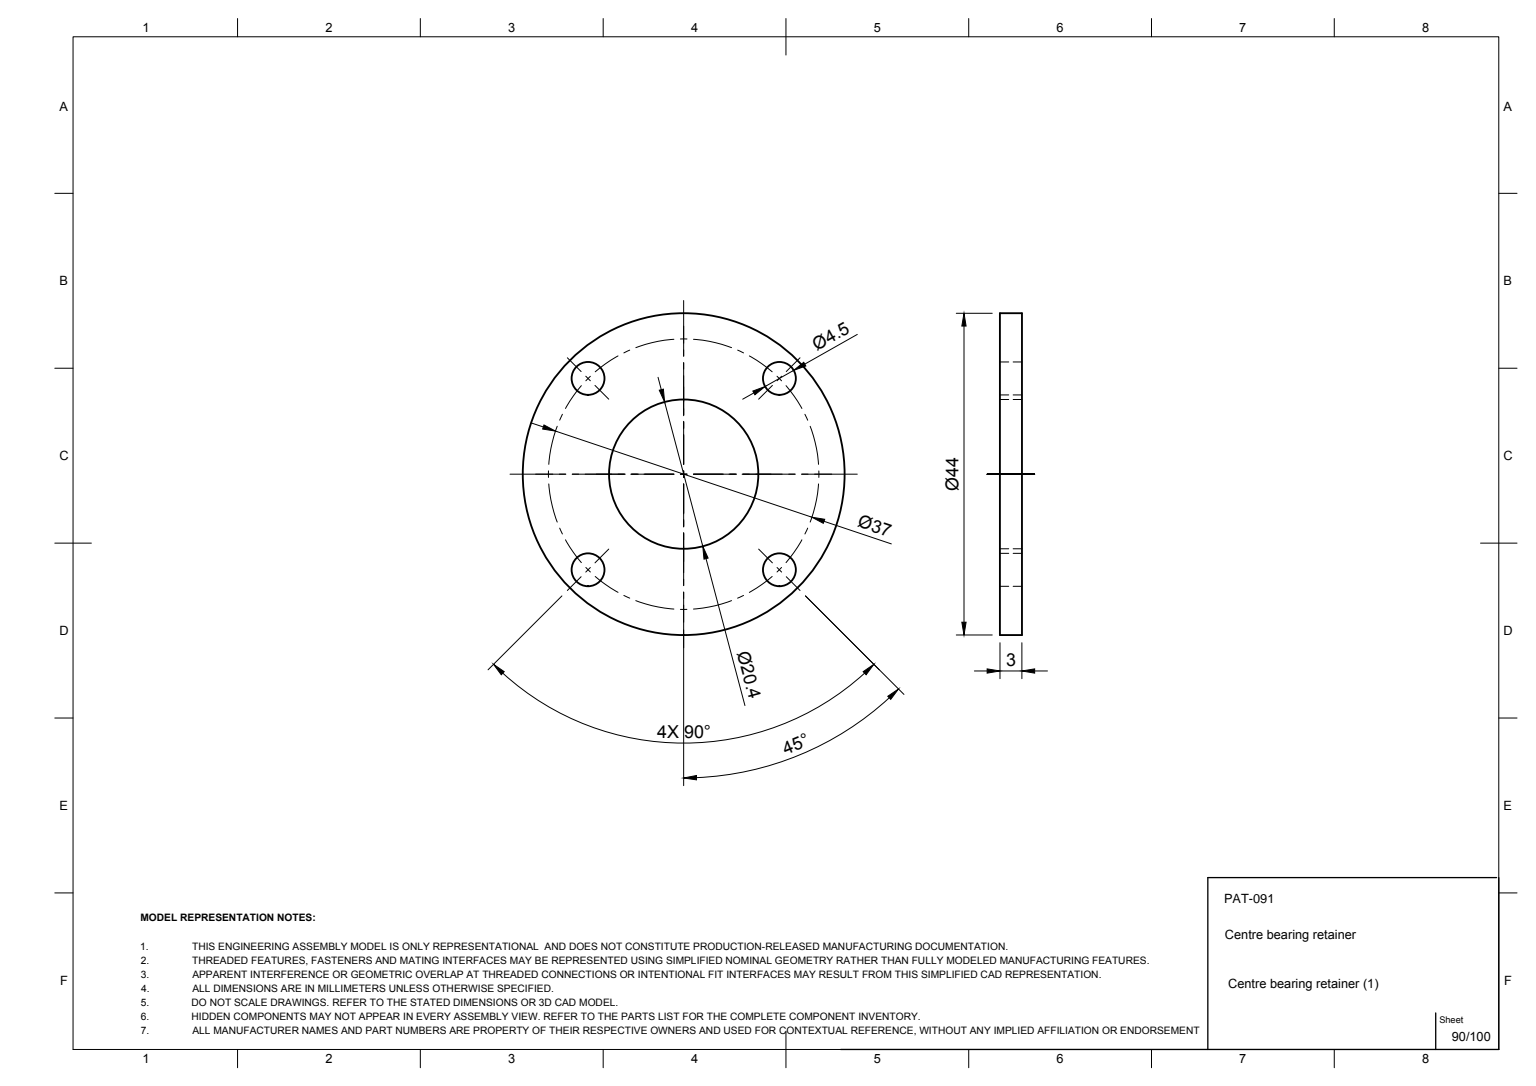
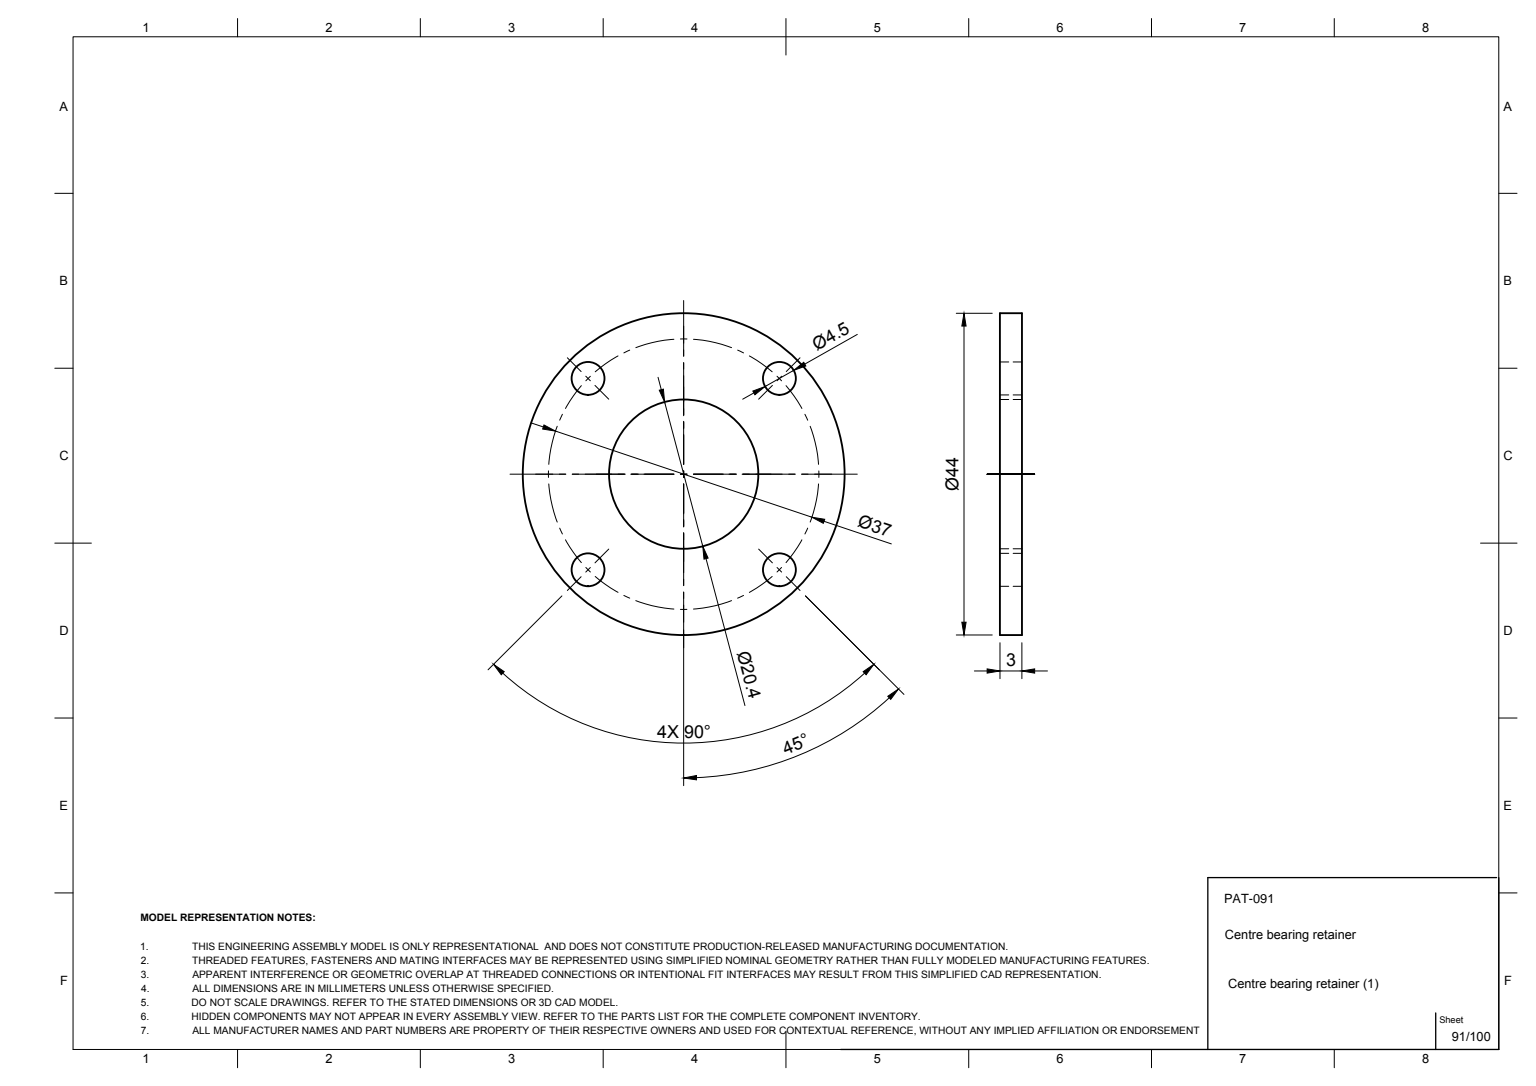
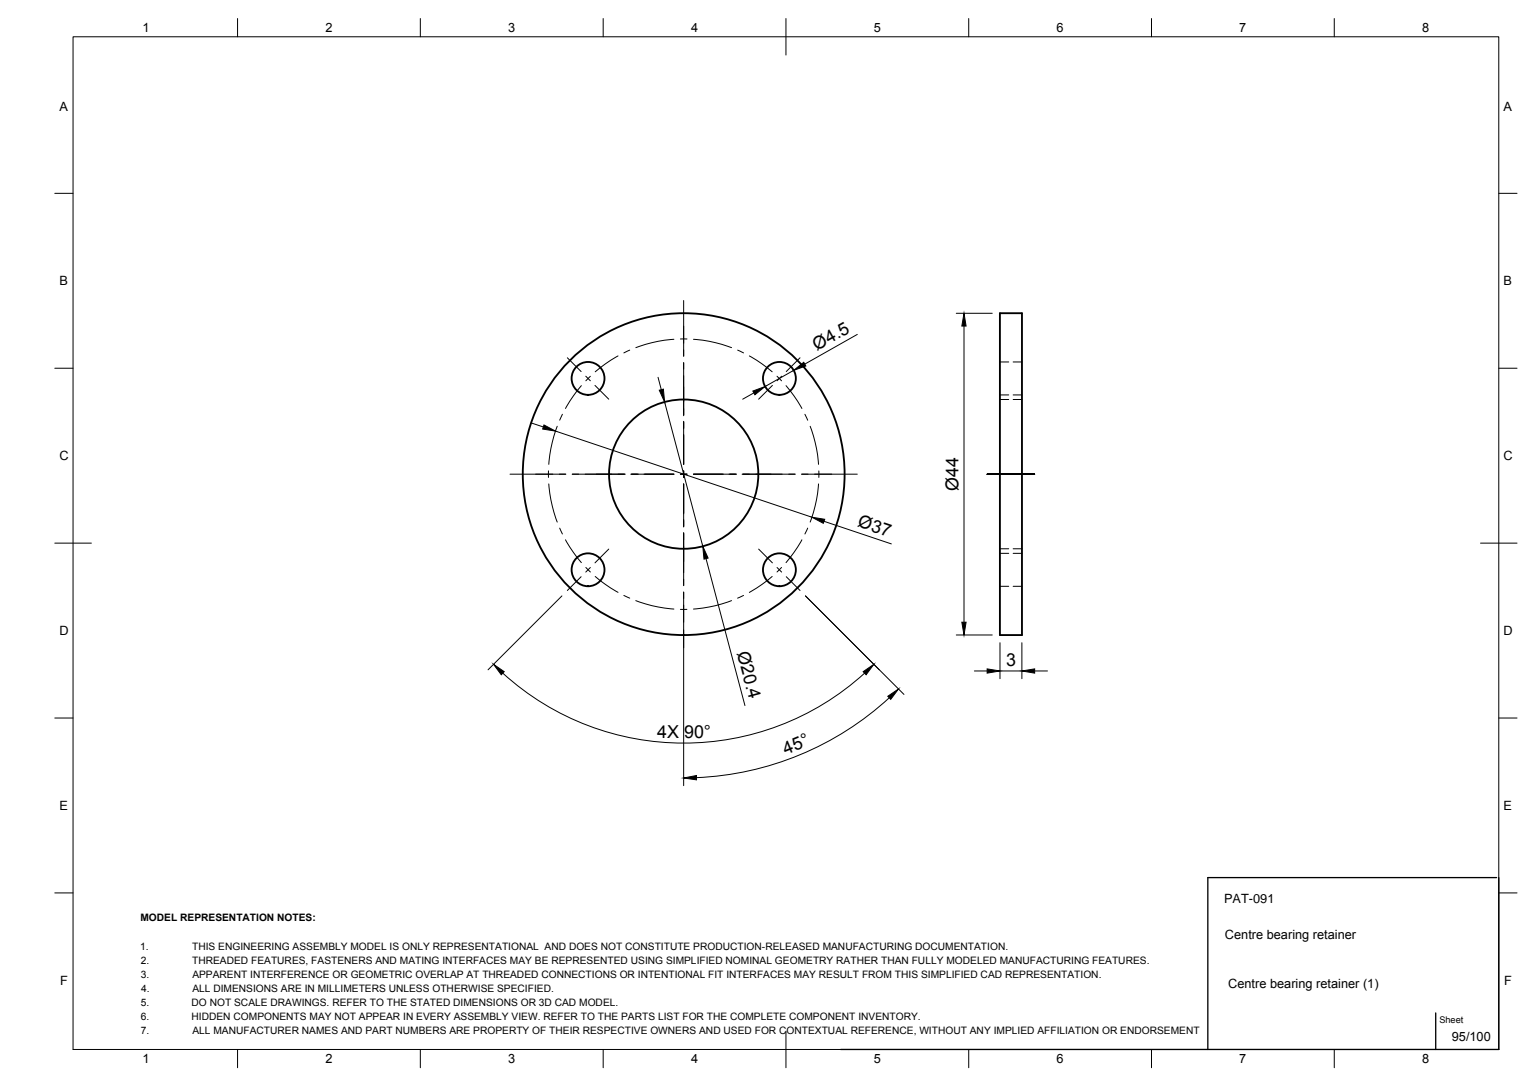
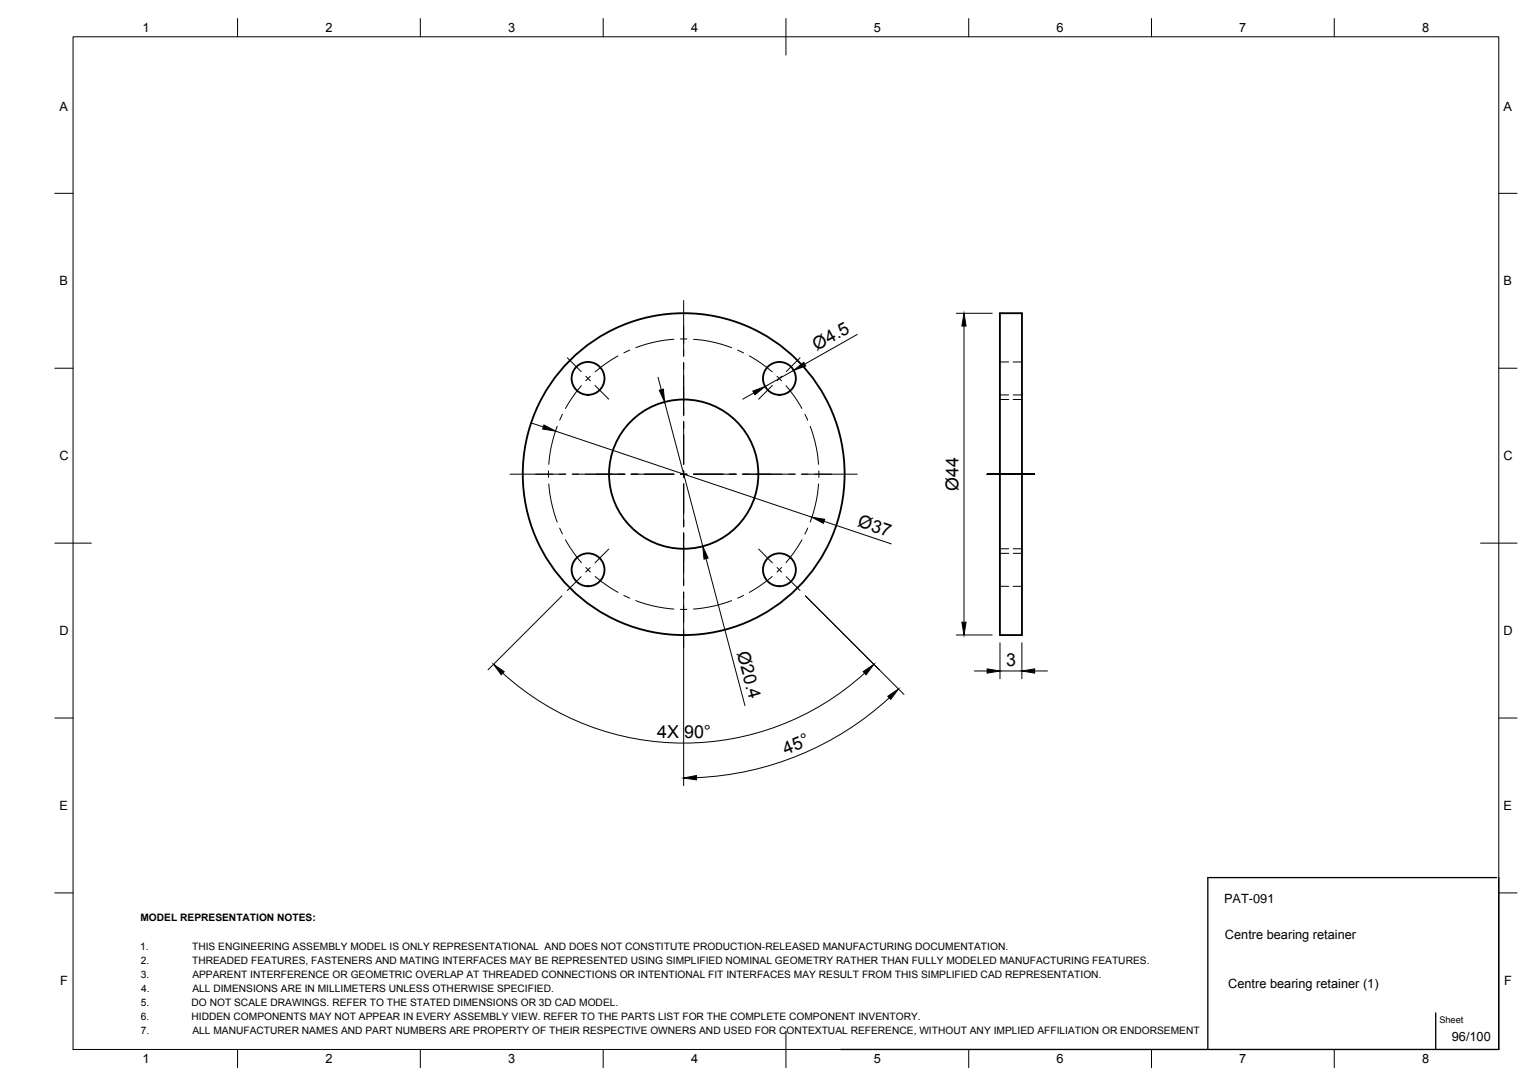
ISO-10303-21;
HEADER;
/* Generated by software containing ST-Developer
 * from STEP Tools, Inc. (www.steptools.com) 
 */

FILE_DESCRIPTION(
/* description */ ('PAT-091'),
/* implementation_level */ '2;1');

FILE_NAME(
/* name */ 'Centre bearing retainer.step',
/* time_stamp */ '2026-10-27T15:34:44-07:00',
/* author */ (''),
/* organization */ (''),
/* preprocessor_version */ 'ST-DEVELOPER v20.2',
/* originating_system */ 'Autodesk Translation Framework v15.17.0.0',
/* authorisation */ '');

FILE_SCHEMA (('AUTOMOTIVE_DESIGN { 1 0 10303 214 3 1 1 }'));
ENDSEC;

DATA;
#10=MECHANICAL_DESIGN_GEOMETRIC_PRESENTATION_REPRESENTATION('',(#1047),#25100);
#827=SHAPE_REPRESENTATION_RELATIONSHIP('SRR','None',#25594,#937);
#937=ADVANCED_BREP_SHAPE_REPRESENTATION('',(#1168),#25064);
#1047=STYLED_ITEM('',(#26191),#1168);
#1168=MANIFOLD_SOLID_BREP('Body1',#13327);
#1543=FACE_BOUND('',#3791,.T.);
#1544=FACE_BOUND('',#3792,.T.);
#1545=FACE_BOUND('',#3793,.T.);
#1546=FACE_BOUND('',#3794,.T.);
#1547=FACE_BOUND('',#3795,.T.);
#1548=FACE_BOUND('',#3797,.T.);
#1549=FACE_BOUND('',#3798,.T.);
#1550=FACE_BOUND('',#3799,.T.);
#1551=FACE_BOUND('',#3800,.T.);
#1552=FACE_BOUND('',#3801,.T.);
#1958=PLANE('',#15849);
#1959=PLANE('',#15850);
#2638=FACE_OUTER_BOUND('',#3784,.T.);
#2639=FACE_OUTER_BOUND('',#3785,.T.);
#2640=FACE_OUTER_BOUND('',#3786,.T.);
#2641=FACE_OUTER_BOUND('',#3787,.T.);
#2642=FACE_OUTER_BOUND('',#3788,.T.);
#2643=FACE_OUTER_BOUND('',#3789,.T.);
#2644=FACE_OUTER_BOUND('',#3790,.T.);
#2645=FACE_OUTER_BOUND('',#3796,.T.);
#3784=EDGE_LOOP('',(#11258,#11259,#11260,#11261));
#3785=EDGE_LOOP('',(#11262,#11263,#11264,#11265));
#3786=EDGE_LOOP('',(#11266,#11267,#11268,#11269));
#3787=EDGE_LOOP('',(#11270,#11271,#11272,#11273));
#3788=EDGE_LOOP('',(#11274,#11275,#11276,#11277));
#3789=EDGE_LOOP('',(#11278,#11279,#11280,#11281));
#3790=EDGE_LOOP('',(#11282));
#3791=EDGE_LOOP('',(#11283));
#3792=EDGE_LOOP('',(#11284));
#3793=EDGE_LOOP('',(#11285));
#3794=EDGE_LOOP('',(#11286));
#3795=EDGE_LOOP('',(#11287));
#3796=EDGE_LOOP('',(#11288));
#3797=EDGE_LOOP('',(#11289));
#3798=EDGE_LOOP('',(#11290));
#3799=EDGE_LOOP('',(#11291));
#3800=EDGE_LOOP('',(#11292));
#3801=EDGE_LOOP('',(#11293));
#4751=LINE('',#23665,#5491);
#4752=LINE('',#23671,#5492);
#4753=LINE('',#23677,#5493);
#4754=LINE('',#23683,#5494);
#4755=LINE('',#23689,#5495);
#4756=LINE('',#23695,#5496);
#5491=VECTOR('',#19591,0.225000000000001);
#5492=VECTOR('',#19598,0.225000000000001);
#5493=VECTOR('',#19605,0.225000000000001);
#5494=VECTOR('',#19612,0.225000000000001);
#5495=VECTOR('',#19619,1.02);
#5496=VECTOR('',#19626,2.2);
#6116=CIRCLE('',#15832,0.225000000000001);
#6117=CIRCLE('',#15833,0.225000000000001);
#6118=CIRCLE('',#15835,0.225000000000001);
#6119=CIRCLE('',#15836,0.225000000000001);
#6120=CIRCLE('',#15838,0.225000000000001);
#6121=CIRCLE('',#15839,0.225000000000001);
#6122=CIRCLE('',#15841,0.225000000000001);
#6123=CIRCLE('',#15842,0.225000000000001);
#6124=CIRCLE('',#15844,1.02);
#6125=CIRCLE('',#15845,1.02);
#6126=CIRCLE('',#15847,2.2);
#6127=CIRCLE('',#15848,2.2);
#7141=VERTEX_POINT('',#23662);
#7142=VERTEX_POINT('',#23664);
#7143=VERTEX_POINT('',#23668);
#7144=VERTEX_POINT('',#23670);
#7145=VERTEX_POINT('',#23674);
#7146=VERTEX_POINT('',#23676);
#7147=VERTEX_POINT('',#23680);
#7148=VERTEX_POINT('',#23682);
#7149=VERTEX_POINT('',#23686);
#7150=VERTEX_POINT('',#23688);
#7151=VERTEX_POINT('',#23692);
#7152=VERTEX_POINT('',#23694);
#8564=EDGE_CURVE('',#7141,#7141,#6116,.T.);
#8565=EDGE_CURVE('',#7141,#7142,#4751,.T.);
#8566=EDGE_CURVE('',#7142,#7142,#6117,.T.);
#8567=EDGE_CURVE('',#7143,#7143,#6118,.T.);
#8568=EDGE_CURVE('',#7143,#7144,#4752,.T.);
#8569=EDGE_CURVE('',#7144,#7144,#6119,.T.);
#8570=EDGE_CURVE('',#7145,#7145,#6120,.T.);
#8571=EDGE_CURVE('',#7145,#7146,#4753,.T.);
#8572=EDGE_CURVE('',#7146,#7146,#6121,.T.);
#8573=EDGE_CURVE('',#7147,#7147,#6122,.T.);
#8574=EDGE_CURVE('',#7147,#7148,#4754,.T.);
#8575=EDGE_CURVE('',#7148,#7148,#6123,.T.);
#8576=EDGE_CURVE('',#7149,#7149,#6124,.T.);
#8577=EDGE_CURVE('',#7149,#7150,#4755,.T.);
#8578=EDGE_CURVE('',#7150,#7150,#6125,.T.);
#8579=EDGE_CURVE('',#7151,#7151,#6126,.T.);
#8580=EDGE_CURVE('',#7151,#7152,#4756,.T.);
#8581=EDGE_CURVE('',#7152,#7152,#6127,.T.);
#11258=ORIENTED_EDGE('',*,*,#8564,.F.);
#11259=ORIENTED_EDGE('',*,*,#8565,.T.);
#11260=ORIENTED_EDGE('',*,*,#8566,.F.);
#11261=ORIENTED_EDGE('',*,*,#8565,.F.);
#11262=ORIENTED_EDGE('',*,*,#8567,.F.);
#11263=ORIENTED_EDGE('',*,*,#8568,.T.);
#11264=ORIENTED_EDGE('',*,*,#8569,.F.);
#11265=ORIENTED_EDGE('',*,*,#8568,.F.);
#11266=ORIENTED_EDGE('',*,*,#8570,.F.);
#11267=ORIENTED_EDGE('',*,*,#8571,.T.);
#11268=ORIENTED_EDGE('',*,*,#8572,.F.);
#11269=ORIENTED_EDGE('',*,*,#8571,.F.);
#11270=ORIENTED_EDGE('',*,*,#8573,.F.);
#11271=ORIENTED_EDGE('',*,*,#8574,.T.);
#11272=ORIENTED_EDGE('',*,*,#8575,.F.);
#11273=ORIENTED_EDGE('',*,*,#8574,.F.);
#11274=ORIENTED_EDGE('',*,*,#8576,.F.);
#11275=ORIENTED_EDGE('',*,*,#8577,.T.);
#11276=ORIENTED_EDGE('',*,*,#8578,.T.);
#11277=ORIENTED_EDGE('',*,*,#8577,.F.);
#11278=ORIENTED_EDGE('',*,*,#8579,.F.);
#11279=ORIENTED_EDGE('',*,*,#8580,.T.);
#11280=ORIENTED_EDGE('',*,*,#8581,.T.);
#11281=ORIENTED_EDGE('',*,*,#8580,.F.);
#11282=ORIENTED_EDGE('',*,*,#8579,.T.);
#11283=ORIENTED_EDGE('',*,*,#8576,.T.);
#11284=ORIENTED_EDGE('',*,*,#8575,.T.);
#11285=ORIENTED_EDGE('',*,*,#8572,.T.);
#11286=ORIENTED_EDGE('',*,*,#8569,.T.);
#11287=ORIENTED_EDGE('',*,*,#8566,.T.);
#11288=ORIENTED_EDGE('',*,*,#8581,.F.);
#11289=ORIENTED_EDGE('',*,*,#8578,.F.);
#11290=ORIENTED_EDGE('',*,*,#8573,.T.);
#11291=ORIENTED_EDGE('',*,*,#8570,.T.);
#11292=ORIENTED_EDGE('',*,*,#8567,.T.);
#11293=ORIENTED_EDGE('',*,*,#8564,.T.);
#12319=CYLINDRICAL_SURFACE('',#15831,0.225000000000001);
#12320=CYLINDRICAL_SURFACE('',#15834,0.225000000000001);
#12321=CYLINDRICAL_SURFACE('',#15837,0.225000000000001);
#12322=CYLINDRICAL_SURFACE('',#15840,0.225000000000001);
#12323=CYLINDRICAL_SURFACE('',#15843,1.02);
#12324=CYLINDRICAL_SURFACE('',#15846,2.2);
#13005=ADVANCED_FACE('',(#2638),#12319,.F.);
#13006=ADVANCED_FACE('',(#2639),#12320,.F.);
#13007=ADVANCED_FACE('',(#2640),#12321,.F.);
#13008=ADVANCED_FACE('',(#2641),#12322,.F.);
#13009=ADVANCED_FACE('',(#2642),#12323,.F.);
#13010=ADVANCED_FACE('',(#2643),#12324,.T.);
#13011=ADVANCED_FACE('',(#2644,#1543,#1544,#1545,#1546,#1547),#1958,.T.);
#13012=ADVANCED_FACE('',(#2645,#1548,#1549,#1550,#1551,#1552),#1959,.F.);
#13327=CLOSED_SHELL('',(#13005,#13006,#13007,#13008,#13009,#13010,#13011,
#13012));
#15830=AXIS2_PLACEMENT_3D('',#23660,#19585,#19586);
#15831=AXIS2_PLACEMENT_3D('',#23661,#19587,#19588);
#15832=AXIS2_PLACEMENT_3D('',#23663,#19589,#19590);
#15833=AXIS2_PLACEMENT_3D('',#23666,#19592,#19593);
#15834=AXIS2_PLACEMENT_3D('',#23667,#19594,#19595);
#15835=AXIS2_PLACEMENT_3D('',#23669,#19596,#19597);
#15836=AXIS2_PLACEMENT_3D('',#23672,#19599,#19600);
#15837=AXIS2_PLACEMENT_3D('',#23673,#19601,#19602);
#15838=AXIS2_PLACEMENT_3D('',#23675,#19603,#19604);
#15839=AXIS2_PLACEMENT_3D('',#23678,#19606,#19607);
#15840=AXIS2_PLACEMENT_3D('',#23679,#19608,#19609);
#15841=AXIS2_PLACEMENT_3D('',#23681,#19610,#19611);
#15842=AXIS2_PLACEMENT_3D('',#23684,#19613,#19614);
#15843=AXIS2_PLACEMENT_3D('',#23685,#19615,#19616);
#15844=AXIS2_PLACEMENT_3D('',#23687,#19617,#19618);
#15845=AXIS2_PLACEMENT_3D('',#23690,#19620,#19621);
#15846=AXIS2_PLACEMENT_3D('',#23691,#19622,#19623);
#15847=AXIS2_PLACEMENT_3D('',#23693,#19624,#19625);
#15848=AXIS2_PLACEMENT_3D('',#23696,#19627,#19628);
#15849=AXIS2_PLACEMENT_3D('',#23697,#19629,#19630);
#15850=AXIS2_PLACEMENT_3D('',#23698,#19631,#19632);
#19585=DIRECTION('axis',(0.,0.,1.));
#19586=DIRECTION('refdir',(1.,0.,0.));
#19587=DIRECTION('center_axis',(0.,1.,0.));
#19588=DIRECTION('ref_axis',(1.,0.,0.));
#19589=DIRECTION('center_axis',(0.,1.,0.));
#19590=DIRECTION('ref_axis',(1.,0.,0.));
#19591=DIRECTION('',(0.,1.,0.));
#19592=DIRECTION('center_axis',(0.,-1.,0.));
#19593=DIRECTION('ref_axis',(1.,0.,0.));
#19594=DIRECTION('center_axis',(0.,1.,0.));
#19595=DIRECTION('ref_axis',(1.,0.,0.));
#19596=DIRECTION('center_axis',(0.,1.,0.));
#19597=DIRECTION('ref_axis',(1.,0.,0.));
#19598=DIRECTION('',(0.,1.,0.));
#19599=DIRECTION('center_axis',(0.,-1.,0.));
#19600=DIRECTION('ref_axis',(1.,0.,0.));
#19601=DIRECTION('center_axis',(0.,1.,0.));
#19602=DIRECTION('ref_axis',(1.,0.,0.));
#19603=DIRECTION('center_axis',(0.,1.,0.));
#19604=DIRECTION('ref_axis',(1.,0.,0.));
#19605=DIRECTION('',(0.,1.,0.));
#19606=DIRECTION('center_axis',(0.,-1.,0.));
#19607=DIRECTION('ref_axis',(1.,0.,0.));
#19608=DIRECTION('center_axis',(0.,1.,0.));
#19609=DIRECTION('ref_axis',(1.,0.,0.));
#19610=DIRECTION('center_axis',(0.,1.,0.));
#19611=DIRECTION('ref_axis',(1.,0.,0.));
#19612=DIRECTION('',(0.,1.,0.));
#19613=DIRECTION('center_axis',(0.,-1.,0.));
#19614=DIRECTION('ref_axis',(1.,0.,0.));
#19615=DIRECTION('center_axis',(0.,1.,0.));
#19616=DIRECTION('ref_axis',(1.,0.,0.));
#19617=DIRECTION('center_axis',(0.,-1.,0.));
#19618=DIRECTION('ref_axis',(1.,0.,0.));
#19619=DIRECTION('',(0.,-1.,0.));
#19620=DIRECTION('center_axis',(0.,-1.,0.));
#19621=DIRECTION('ref_axis',(1.,0.,0.));
#19622=DIRECTION('center_axis',(0.,1.,0.));
#19623=DIRECTION('ref_axis',(1.,0.,0.));
#19624=DIRECTION('center_axis',(0.,1.,0.));
#19625=DIRECTION('ref_axis',(1.,0.,0.));
#19626=DIRECTION('',(0.,-1.,0.));
#19627=DIRECTION('center_axis',(0.,1.,0.));
#19628=DIRECTION('ref_axis',(1.,0.,0.));
#19629=DIRECTION('center_axis',(0.,1.,0.));
#19630=DIRECTION('ref_axis',(1.,0.,0.));
#19631=DIRECTION('center_axis',(0.,1.,0.));
#19632=DIRECTION('ref_axis',(1.,0.,0.));
#23660=CARTESIAN_POINT('',(0.,0.,0.));
#23661=CARTESIAN_POINT('Origin',(18.056769185842,-5.9,6.69185245480489));
#23662=CARTESIAN_POINT('',(17.831769185842,-5.8,6.69185245480489));
#23663=CARTESIAN_POINT('Origin',(18.056769185842,-5.8,6.69185245480489));
#23664=CARTESIAN_POINT('',(17.831769185842,-5.5,6.69185245480489));
#23665=CARTESIAN_POINT('',(17.831769185842,-5.9,6.69185245480489));
#23666=CARTESIAN_POINT('Origin',(18.056769185842,-5.5,6.69185245480489));
#23667=CARTESIAN_POINT('Origin',(18.056769185842,-5.9,9.30814754519511));
#23668=CARTESIAN_POINT('',(17.831769185842,-5.8,9.30814754519511));
#23669=CARTESIAN_POINT('Origin',(18.056769185842,-5.8,9.30814754519511));
#23670=CARTESIAN_POINT('',(17.831769185842,-5.5,9.30814754519511));
#23671=CARTESIAN_POINT('',(17.831769185842,-5.9,9.30814754519511));
#23672=CARTESIAN_POINT('Origin',(18.056769185842,-5.5,9.30814754519511));
#23673=CARTESIAN_POINT('Origin',(20.6730642762322,-5.9,9.30814754519511));
#23674=CARTESIAN_POINT('',(20.4480642762322,-5.8,9.30814754519511));
#23675=CARTESIAN_POINT('Origin',(20.6730642762322,-5.8,9.30814754519511));
#23676=CARTESIAN_POINT('',(20.4480642762322,-5.5,9.30814754519511));
#23677=CARTESIAN_POINT('',(20.4480642762322,-5.9,9.30814754519511));
#23678=CARTESIAN_POINT('Origin',(20.6730642762322,-5.5,9.30814754519511));
#23679=CARTESIAN_POINT('Origin',(20.6730642762322,-5.9,6.69185245480489));
#23680=CARTESIAN_POINT('',(20.4480642762322,-5.8,6.69185245480489));
#23681=CARTESIAN_POINT('Origin',(20.6730642762322,-5.8,6.69185245480489));
#23682=CARTESIAN_POINT('',(20.4480642762322,-5.5,6.69185245480489));
#23683=CARTESIAN_POINT('',(20.4480642762322,-5.9,6.69185245480489));
#23684=CARTESIAN_POINT('Origin',(20.6730642762322,-5.5,6.69185245480489));
#23685=CARTESIAN_POINT('Origin',(19.3649167310371,-5.8,8.));
#23686=CARTESIAN_POINT('',(18.3449167310371,-5.5,8.));
#23687=CARTESIAN_POINT('Origin',(19.3649167310371,-5.5,8.));
#23688=CARTESIAN_POINT('',(18.3449167310371,-5.8,8.));
#23689=CARTESIAN_POINT('',(18.3449167310371,-5.8,8.));
#23690=CARTESIAN_POINT('Origin',(19.3649167310371,-5.8,8.));
#23691=CARTESIAN_POINT('Origin',(19.3649167310371,-5.8,8.));
#23692=CARTESIAN_POINT('',(17.1649167310371,-5.5,8.));
#23693=CARTESIAN_POINT('Origin',(19.3649167310371,-5.5,8.));
#23694=CARTESIAN_POINT('',(17.1649167310371,-5.8,8.));
#23695=CARTESIAN_POINT('',(17.1649167310371,-5.8,8.));
#23696=CARTESIAN_POINT('Origin',(19.3649167310371,-5.8,8.));
#23697=CARTESIAN_POINT('Origin',(19.3649167310371,-5.5,8.));
#23698=CARTESIAN_POINT('Origin',(19.3649167310371,-5.8,8.));
#24943=UNCERTAINTY_MEASURE_WITH_UNIT(LENGTH_MEASURE(0.001),#25101,
'DISTANCE_ACCURACY_VALUE',
'Maximum model space distance between geometric entities at asserted c
onnectivities');
#24979=UNCERTAINTY_MEASURE_WITH_UNIT(LENGTH_MEASURE(0.001),#25101,
'DISTANCE_ACCURACY_VALUE',
'Maximum model space distance between geometric entities at asserted c
onnectivities');
#25064=(
GEOMETRIC_REPRESENTATION_CONTEXT(3)
GLOBAL_UNCERTAINTY_ASSIGNED_CONTEXT((#24943))
GLOBAL_UNIT_ASSIGNED_CONTEXT((#25101,#25103,#25104))
REPRESENTATION_CONTEXT('','3D')
);
#25100=(
GEOMETRIC_REPRESENTATION_CONTEXT(3)
GLOBAL_UNCERTAINTY_ASSIGNED_CONTEXT((#24979))
GLOBAL_UNIT_ASSIGNED_CONTEXT((#25101,#25103,#25104))
REPRESENTATION_CONTEXT('','3D')
);
#25101=(
LENGTH_UNIT()
NAMED_UNIT(*)
SI_UNIT(.CENTI.,.METRE.)
);
#25103=(
NAMED_UNIT(*)
PLANE_ANGLE_UNIT()
SI_UNIT($,.RADIAN.)
);
#25104=(
NAMED_UNIT(*)
SI_UNIT($,.STERADIAN.)
SOLID_ANGLE_UNIT()
);
#25189=SHAPE_DEFINITION_REPRESENTATION(#25383,#25594);
#25383=PRODUCT_DEFINITION_SHAPE('',$,#25715);
#25594=SHAPE_REPRESENTATION('',(#15830),#25064);
#25630=PRODUCT_DEFINITION_CONTEXT('part definition',#25992,'design');
#25715=PRODUCT_DEFINITION('Centre bearing retainer',
'Centre bearing retainer',#25835,#25630);
#25835=PRODUCT_DEFINITION_FORMATION('',$,#26078);
#25992=APPLICATION_CONTEXT(
'Core Data for Automotive Mechanical Design Process');
#25993=PRODUCT_CONTEXT('part definition',#25992,'mechanical');
#26078=PRODUCT('Centre bearing retainer','Centre bearing retainer',
'Centre bearing retainer',(#25993));
#26185=COLOUR_RGB('Grey',0.48,0.52,0.57);
#26186=FILL_AREA_STYLE_COLOUR('',#26185);
#26187=FILL_AREA_STYLE('',(#26186));
#26188=SURFACE_STYLE_FILL_AREA(#26187);
#26189=SURFACE_SIDE_STYLE('',(#26188));
#26190=SURFACE_STYLE_USAGE(.BOTH.,#26189);
#26191=PRESENTATION_STYLE_ASSIGNMENT((#26190));
ENDSEC;
END-ISO-10303-21;
